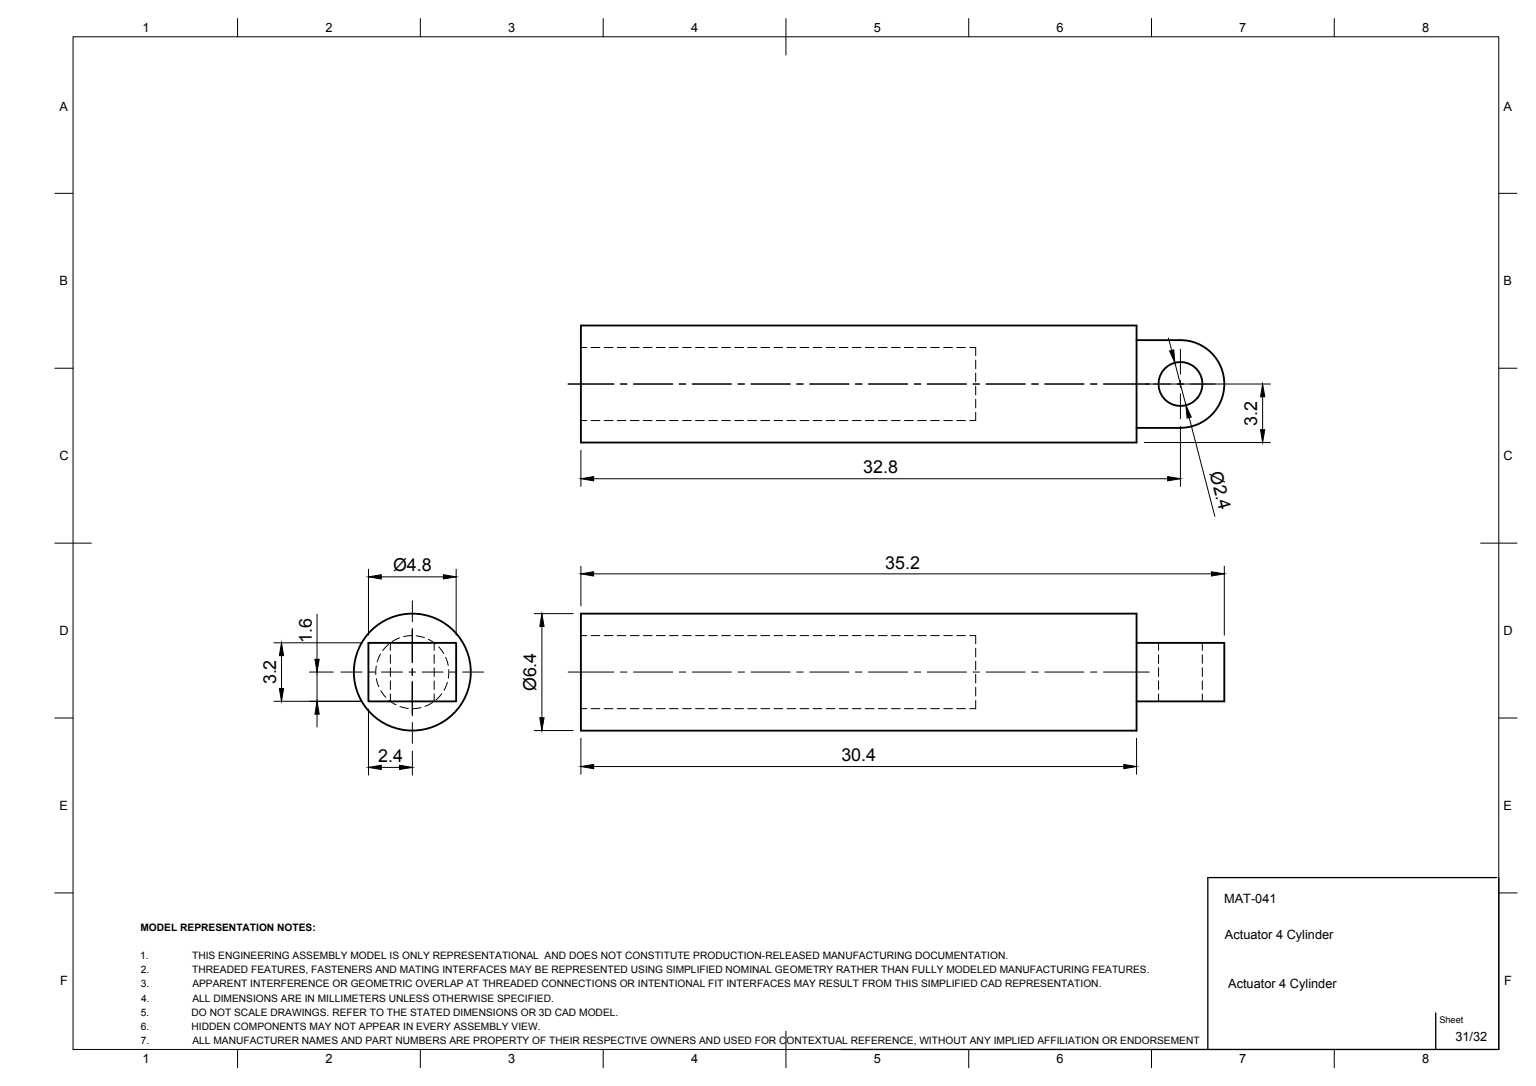
ISO-10303-21;
HEADER;
/* Generated by software containing ST-Developer
 * from STEP Tools, Inc. (www.steptools.com) 
 */

FILE_DESCRIPTION(
/* description */ ('STEP AP214'),
/* implementation_level */ '2;1');

FILE_NAME(
/* name */ 'Actuator 4 Cylinder.step',
/* time_stamp */ '2026-11-14T21:57:47-08:00',
/* author */ (''),
/* organization */ (''),
/* preprocessor_version */ 'ST-DEVELOPER v20.2',
/* originating_system */ 'Autodesk Translation Framework v15.17.0.0',
/* authorisation */ '');

FILE_SCHEMA (('AUTOMOTIVE_DESIGN { 1 0 10303 214 3 1 1 }'));
ENDSEC;

DATA;
#10=MECHANICAL_DESIGN_GEOMETRIC_PRESENTATION_REPRESENTATION('',(#264),#13199);
#228=SHAPE_REPRESENTATION_RELATIONSHIP('SRR','None',#13301,#246);
#246=ADVANCED_BREP_SHAPE_REPRESENTATION('',(#282),#13197);
#264=STYLED_ITEM('',(#13409),#282);
#282=MANIFOLD_SOLID_BREP('Body1',#6859);
#376=FACE_BOUND('',#2658,.T.);
#377=FACE_BOUND('',#2660,.T.);
#378=FACE_BOUND('',#2662,.T.);
#379=FACE_BOUND('',#2665,.T.);
#597=PLANE('',#7793);
#598=PLANE('',#7794);
#599=PLANE('',#7795);
#600=PLANE('',#7797);
#601=PLANE('',#7798);
#602=PLANE('',#7800);
#603=PLANE('',#7802);
#1103=LINE('',#13056,#1621);
#1104=LINE('',#13062,#1622);
#1105=LINE('',#13068,#1623);
#1106=LINE('',#13073,#1624);
#1107=LINE('',#13075,#1625);
#1108=LINE('',#13077,#1626);
#1109=LINE('',#13078,#1627);
#1110=LINE('',#13084,#1628);
#1111=LINE('',#13085,#1629);
#1112=LINE('',#13088,#1630);
#1113=LINE('',#13089,#1631);
#1114=LINE('',#13092,#1632);
#1115=LINE('',#13095,#1633);
#1621=VECTOR('',#9774,2.);
#1622=VECTOR('',#9781,1.2);
#1623=VECTOR('',#9788,3.2);
#1624=VECTOR('',#9793,1000.);
#1625=VECTOR('',#9794,1000.);
#1626=VECTOR('',#9795,1000.);
#1627=VECTOR('',#9796,1000.);
#1628=VECTOR('',#9803,1000.);
#1629=VECTOR('',#9804,1000.);
#1630=VECTOR('',#9807,1000.);
#1631=VECTOR('',#9808,1000.);
#1632=VECTOR('',#9811,1000.);
#1633=VECTOR('',#9816,1000.);
#1782=CYLINDRICAL_SURFACE('',#7784,2.);
#1783=CYLINDRICAL_SURFACE('',#7787,1.2);
#1784=CYLINDRICAL_SURFACE('',#7790,3.2);
#1785=CYLINDRICAL_SURFACE('',#7801,2.4);
#2171=FACE_OUTER_BOUND('',#2654,.T.);
#2172=FACE_OUTER_BOUND('',#2655,.T.);
#2173=FACE_OUTER_BOUND('',#2656,.T.);
#2174=FACE_OUTER_BOUND('',#2657,.T.);
#2175=FACE_OUTER_BOUND('',#2659,.T.);
#2176=FACE_OUTER_BOUND('',#2661,.T.);
#2177=FACE_OUTER_BOUND('',#2663,.T.);
#2178=FACE_OUTER_BOUND('',#2664,.T.);
#2179=FACE_OUTER_BOUND('',#2666,.T.);
#2180=FACE_OUTER_BOUND('',#2667,.T.);
#2181=FACE_OUTER_BOUND('',#2668,.T.);
#2654=EDGE_LOOP('',(#6364,#6365,#6366,#6367));
#2655=EDGE_LOOP('',(#6368,#6369,#6370,#6371));
#2656=EDGE_LOOP('',(#6372,#6373,#6374,#6375));
#2657=EDGE_LOOP('',(#6376));
#2658=EDGE_LOOP('',(#6377,#6378,#6379,#6380));
#2659=EDGE_LOOP('',(#6381));
#2660=EDGE_LOOP('',(#6382));
#2661=EDGE_LOOP('',(#6383,#6384,#6385,#6386));
#2662=EDGE_LOOP('',(#6387));
#2663=EDGE_LOOP('',(#6388,#6389,#6390,#6391));
#2664=EDGE_LOOP('',(#6392,#6393,#6394,#6395));
#2665=EDGE_LOOP('',(#6396));
#2666=EDGE_LOOP('',(#6397,#6398,#6399,#6400));
#2667=EDGE_LOOP('',(#6401,#6402,#6403,#6404));
#2668=EDGE_LOOP('',(#6405));
#2986=CIRCLE('',#7785,2.);
#2987=CIRCLE('',#7786,2.);
#2988=CIRCLE('',#7788,1.2);
#2989=CIRCLE('',#7789,1.2);
#2990=CIRCLE('',#7791,3.2);
#2991=CIRCLE('',#7792,3.2);
#2992=CIRCLE('',#7796,2.4);
#2993=CIRCLE('',#7799,2.4);
#3590=VERTEX_POINT('',#13053);
#3591=VERTEX_POINT('',#13055);
#3592=VERTEX_POINT('',#13059);
#3593=VERTEX_POINT('',#13061);
#3594=VERTEX_POINT('',#13065);
#3595=VERTEX_POINT('',#13067);
#3596=VERTEX_POINT('',#13071);
#3597=VERTEX_POINT('',#13072);
#3598=VERTEX_POINT('',#13074);
#3599=VERTEX_POINT('',#13076);
#3600=VERTEX_POINT('',#13081);
#3601=VERTEX_POINT('',#13082);
#3602=VERTEX_POINT('',#13087);
#3603=VERTEX_POINT('',#13091);
#4519=EDGE_CURVE('',#3590,#3590,#2986,.T.);
#4520=EDGE_CURVE('',#3590,#3591,#1103,.T.);
#4521=EDGE_CURVE('',#3591,#3591,#2987,.T.);
#4522=EDGE_CURVE('',#3592,#3592,#2988,.T.);
#4523=EDGE_CURVE('',#3592,#3593,#1104,.T.);
#4524=EDGE_CURVE('',#3593,#3593,#2989,.T.);
#4525=EDGE_CURVE('',#3594,#3594,#2990,.T.);
#4526=EDGE_CURVE('',#3594,#3595,#1105,.T.);
#4527=EDGE_CURVE('',#3595,#3595,#2991,.T.);
#4528=EDGE_CURVE('',#3596,#3597,#1106,.T.);
#4529=EDGE_CURVE('',#3598,#3596,#1107,.T.);
#4530=EDGE_CURVE('',#3599,#3598,#1108,.T.);
#4531=EDGE_CURVE('',#3597,#3599,#1109,.T.);
#4532=EDGE_CURVE('',#3600,#3601,#2992,.T.);
#4533=EDGE_CURVE('',#3601,#3596,#1110,.T.);
#4534=EDGE_CURVE('',#3600,#3597,#1111,.T.);
#4535=EDGE_CURVE('',#3602,#3599,#1112,.T.);
#4536=EDGE_CURVE('',#3602,#3600,#1113,.T.);
#4537=EDGE_CURVE('',#3603,#3598,#1114,.T.);
#4538=EDGE_CURVE('',#3603,#3602,#2993,.T.);
#4539=EDGE_CURVE('',#3601,#3603,#1115,.T.);
#6364=ORIENTED_EDGE('',*,*,#4519,.F.);
#6365=ORIENTED_EDGE('',*,*,#4520,.T.);
#6366=ORIENTED_EDGE('',*,*,#4521,.T.);
#6367=ORIENTED_EDGE('',*,*,#4520,.F.);
#6368=ORIENTED_EDGE('',*,*,#4522,.F.);
#6369=ORIENTED_EDGE('',*,*,#4523,.T.);
#6370=ORIENTED_EDGE('',*,*,#4524,.T.);
#6371=ORIENTED_EDGE('',*,*,#4523,.F.);
#6372=ORIENTED_EDGE('',*,*,#4525,.T.);
#6373=ORIENTED_EDGE('',*,*,#4526,.T.);
#6374=ORIENTED_EDGE('',*,*,#4527,.F.);
#6375=ORIENTED_EDGE('',*,*,#4526,.F.);
#6376=ORIENTED_EDGE('',*,*,#4525,.F.);
#6377=ORIENTED_EDGE('',*,*,#4528,.F.);
#6378=ORIENTED_EDGE('',*,*,#4529,.F.);
#6379=ORIENTED_EDGE('',*,*,#4530,.F.);
#6380=ORIENTED_EDGE('',*,*,#4531,.F.);
#6381=ORIENTED_EDGE('',*,*,#4527,.T.);
#6382=ORIENTED_EDGE('',*,*,#4521,.F.);
#6383=ORIENTED_EDGE('',*,*,#4532,.T.);
#6384=ORIENTED_EDGE('',*,*,#4533,.T.);
#6385=ORIENTED_EDGE('',*,*,#4528,.T.);
#6386=ORIENTED_EDGE('',*,*,#4534,.F.);
#6387=ORIENTED_EDGE('',*,*,#4522,.T.);
#6388=ORIENTED_EDGE('',*,*,#4535,.F.);
#6389=ORIENTED_EDGE('',*,*,#4536,.T.);
#6390=ORIENTED_EDGE('',*,*,#4534,.T.);
#6391=ORIENTED_EDGE('',*,*,#4531,.T.);
#6392=ORIENTED_EDGE('',*,*,#4537,.F.);
#6393=ORIENTED_EDGE('',*,*,#4538,.T.);
#6394=ORIENTED_EDGE('',*,*,#4535,.T.);
#6395=ORIENTED_EDGE('',*,*,#4530,.T.);
#6396=ORIENTED_EDGE('',*,*,#4524,.F.);
#6397=ORIENTED_EDGE('',*,*,#4533,.F.);
#6398=ORIENTED_EDGE('',*,*,#4539,.T.);
#6399=ORIENTED_EDGE('',*,*,#4537,.T.);
#6400=ORIENTED_EDGE('',*,*,#4529,.T.);
#6401=ORIENTED_EDGE('',*,*,#4536,.F.);
#6402=ORIENTED_EDGE('',*,*,#4538,.F.);
#6403=ORIENTED_EDGE('',*,*,#4539,.F.);
#6404=ORIENTED_EDGE('',*,*,#4532,.F.);
#6405=ORIENTED_EDGE('',*,*,#4519,.T.);
#6823=ADVANCED_FACE('',(#2171),#1782,.F.);
#6824=ADVANCED_FACE('',(#2172),#1783,.F.);
#6825=ADVANCED_FACE('',(#2173),#1784,.T.);
#6826=ADVANCED_FACE('',(#2174,#376),#597,.F.);
#6827=ADVANCED_FACE('',(#2175,#377),#598,.T.);
#6828=ADVANCED_FACE('',(#2176,#378),#599,.F.);
#6829=ADVANCED_FACE('',(#2177),#600,.F.);
#6830=ADVANCED_FACE('',(#2178,#379),#601,.F.);
#6831=ADVANCED_FACE('',(#2179),#602,.F.);
#6832=ADVANCED_FACE('',(#2180),#1785,.T.);
#6833=ADVANCED_FACE('',(#2181),#603,.T.);
#6859=CLOSED_SHELL('',(#6823,#6824,#6825,#6826,#6827,#6828,#6829,#6830,
#6831,#6832,#6833));
#7783=AXIS2_PLACEMENT_3D('',#13051,#9768,#9769);
#7784=AXIS2_PLACEMENT_3D('',#13052,#9770,#9771);
#7785=AXIS2_PLACEMENT_3D('',#13054,#9772,#9773);
#7786=AXIS2_PLACEMENT_3D('',#13057,#9775,#9776);
#7787=AXIS2_PLACEMENT_3D('',#13058,#9777,#9778);
#7788=AXIS2_PLACEMENT_3D('',#13060,#9779,#9780);
#7789=AXIS2_PLACEMENT_3D('',#13063,#9782,#9783);
#7790=AXIS2_PLACEMENT_3D('',#13064,#9784,#9785);
#7791=AXIS2_PLACEMENT_3D('',#13066,#9786,#9787);
#7792=AXIS2_PLACEMENT_3D('',#13069,#9789,#9790);
#7793=AXIS2_PLACEMENT_3D('',#13070,#9791,#9792);
#7794=AXIS2_PLACEMENT_3D('',#13079,#9797,#9798);
#7795=AXIS2_PLACEMENT_3D('',#13080,#9799,#9800);
#7796=AXIS2_PLACEMENT_3D('',#13083,#9801,#9802);
#7797=AXIS2_PLACEMENT_3D('',#13086,#9805,#9806);
#7798=AXIS2_PLACEMENT_3D('',#13090,#9809,#9810);
#7799=AXIS2_PLACEMENT_3D('',#13093,#9812,#9813);
#7800=AXIS2_PLACEMENT_3D('',#13094,#9814,#9815);
#7801=AXIS2_PLACEMENT_3D('',#13096,#9817,#9818);
#7802=AXIS2_PLACEMENT_3D('',#13097,#9819,#9820);
#9768=DIRECTION('axis',(0.,0.,1.));
#9769=DIRECTION('refdir',(1.,0.,0.));
#9770=DIRECTION('center_axis',(0.,0.,1.));
#9771=DIRECTION('ref_axis',(1.,0.,0.));
#9772=DIRECTION('center_axis',(0.,0.,1.));
#9773=DIRECTION('ref_axis',(1.,0.,0.));
#9774=DIRECTION('',(0.,0.,1.));
#9775=DIRECTION('center_axis',(0.,0.,1.));
#9776=DIRECTION('ref_axis',(1.,0.,0.));
#9777=DIRECTION('center_axis',(1.,-1.0842021724855E-16,0.));
#9778=DIRECTION('ref_axis',(1.0842021724855E-16,1.,0.));
#9779=DIRECTION('center_axis',(1.,-7.2280144832367E-17,0.));
#9780=DIRECTION('ref_axis',(7.2280144832367E-17,1.,0.));
#9781=DIRECTION('',(1.,-1.0842021724855E-16,0.));
#9782=DIRECTION('center_axis',(1.,-1.0842021724855E-16,0.));
#9783=DIRECTION('ref_axis',(1.0842021724855E-16,1.,0.));
#9784=DIRECTION('center_axis',(0.,0.,-1.));
#9785=DIRECTION('ref_axis',(-1.,0.,0.));
#9786=DIRECTION('center_axis',(0.,0.,1.));
#9787=DIRECTION('ref_axis',(1.,0.,0.));
#9788=DIRECTION('',(0.,0.,1.));
#9789=DIRECTION('center_axis',(0.,0.,1.));
#9790=DIRECTION('ref_axis',(1.,0.,0.));
#9791=DIRECTION('center_axis',(0.,0.,1.));
#9792=DIRECTION('ref_axis',(1.,0.,0.));
#9793=DIRECTION('',(7.2280144832367E-17,1.,0.));
#9794=DIRECTION('',(-1.,0.,0.));
#9795=DIRECTION('',(-1.44560289664734E-16,-1.,0.));
#9796=DIRECTION('',(1.,0.,0.));
#9797=DIRECTION('center_axis',(0.,0.,1.));
#9798=DIRECTION('ref_axis',(1.,0.,0.));
#9799=DIRECTION('center_axis',(1.,-7.2280144832367E-17,0.));
#9800=DIRECTION('ref_axis',(7.2280144832367E-17,1.,0.));
#9801=DIRECTION('center_axis',(-1.,7.2280144832367E-17,0.));
#9802=DIRECTION('ref_axis',(7.2280144832367E-17,1.,0.));
#9803=DIRECTION('',(0.,0.,1.));
#9804=DIRECTION('',(0.,0.,1.));
#9805=DIRECTION('center_axis',(0.,-1.,0.));
#9806=DIRECTION('ref_axis',(0.,0.,-1.));
#9807=DIRECTION('',(0.,0.,1.));
#9808=DIRECTION('',(-1.,0.,0.));
#9809=DIRECTION('center_axis',(-1.,1.44560289664734E-16,0.));
#9810=DIRECTION('ref_axis',(-1.44560289664734E-16,-1.,0.));
#9811=DIRECTION('',(0.,0.,1.));
#9812=DIRECTION('center_axis',(1.,-1.44560289664734E-16,0.));
#9813=DIRECTION('ref_axis',(-1.44560289664734E-16,-1.,0.));
#9814=DIRECTION('center_axis',(0.,1.,0.));
#9815=DIRECTION('ref_axis',(0.,0.,1.));
#9816=DIRECTION('',(1.,0.,0.));
#9817=DIRECTION('center_axis',(-1.,0.,0.));
#9818=DIRECTION('ref_axis',(0.,1.22464679914735E-16,-1.));
#9819=DIRECTION('center_axis',(0.,0.,1.));
#9820=DIRECTION('ref_axis',(1.,0.,0.));
#13051=CARTESIAN_POINT('',(0.,0.,0.));
#13052=CARTESIAN_POINT('Origin',(3.77881193895716E-17,0.,11.9128278522764));
#13053=CARTESIAN_POINT('',(-2.,-2.44929359829471E-16,11.9128278522764));
#13054=CARTESIAN_POINT('Origin',(3.77881193895716E-17,0.,11.9128278522764));
#13055=CARTESIAN_POINT('',(-2.,-2.44929359829471E-16,33.5128278522764));
#13056=CARTESIAN_POINT('',(-2.,-2.44929359829471E-16,11.9128278522764));
#13057=CARTESIAN_POINT('Origin',(3.77881193895716E-17,0.,33.5128278522764));
#13058=CARTESIAN_POINT('Origin',(-3.2,4.19224840027728E-16,0.712827852276406));
#13059=CARTESIAN_POINT('',(-1.6,-1.2,0.712827852276406));
#13060=CARTESIAN_POINT('Origin',(-1.6,2.45752492430048E-16,0.712827852276406));
#13061=CARTESIAN_POINT('',(1.6,-1.2,0.712827852276406));
#13062=CARTESIAN_POINT('',(-3.2,-1.2,0.712827852276406));
#13063=CARTESIAN_POINT('Origin',(1.6,-1.01192202765314E-16,0.712827852276406));
#13064=CARTESIAN_POINT('Origin',(3.77881193895716E-17,0.,33.5128278522764));
#13065=CARTESIAN_POINT('',(3.2,-3.91886975727153E-16,3.11282785227641));
#13066=CARTESIAN_POINT('Origin',(3.77881193895716E-17,0.,3.11282785227641));
#13067=CARTESIAN_POINT('',(3.2,-3.91886975727153E-16,33.5128278522764));
#13068=CARTESIAN_POINT('',(3.2,-3.91886975727153E-16,33.5128278522764));
#13069=CARTESIAN_POINT('Origin',(3.77881193895716E-17,0.,33.5128278522764));
#13070=CARTESIAN_POINT('Origin',(3.77881193895716E-17,0.,3.11282785227641));
#13071=CARTESIAN_POINT('',(-1.6,-2.4,3.11282785227641));
#13072=CARTESIAN_POINT('',(-1.6,2.4,3.11282785227641));
#13073=CARTESIAN_POINT('',(-1.6,2.4,3.11282785227641));
#13074=CARTESIAN_POINT('',(1.6,-2.4,3.11282785227641));
#13075=CARTESIAN_POINT('',(1.6,-2.4,3.11282785227641));
#13076=CARTESIAN_POINT('',(1.6,2.4,3.11282785227641));
#13077=CARTESIAN_POINT('',(1.6,2.4,3.11282785227641));
#13078=CARTESIAN_POINT('',(1.6,2.4,3.11282785227641));
#13079=CARTESIAN_POINT('Origin',(3.77881193895716E-17,0.,33.5128278522764));
#13080=CARTESIAN_POINT('Origin',(-1.6,2.4,-1.68717214772359));
#13081=CARTESIAN_POINT('',(-1.6,2.4,0.712827852276406));
#13082=CARTESIAN_POINT('',(-1.6,-2.4,0.712827852276406));
#13083=CARTESIAN_POINT('Origin',(-1.6,0.,0.712827852276406));
#13084=CARTESIAN_POINT('',(-1.6,-2.4,-1.68717214772359));
#13085=CARTESIAN_POINT('',(-1.6,2.4,-1.68717214772359));
#13086=CARTESIAN_POINT('Origin',(1.6,2.4,-1.68717214772359));
#13087=CARTESIAN_POINT('',(1.6,2.4,0.712827852276406));
#13088=CARTESIAN_POINT('',(1.6,2.4,-1.68717214772359));
#13089=CARTESIAN_POINT('',(-1.6,2.4,0.712827852276406));
#13090=CARTESIAN_POINT('Origin',(1.6,2.4,-1.68717214772359));
#13091=CARTESIAN_POINT('',(1.6,-2.4,0.712827852276406));
#13092=CARTESIAN_POINT('',(1.6,-2.4,-1.68717214772359));
#13093=CARTESIAN_POINT('Origin',(1.6,0.,0.712827852276406));
#13094=CARTESIAN_POINT('Origin',(1.6,-2.4,-1.68717214772359));
#13095=CARTESIAN_POINT('',(1.6,-2.4,0.712827852276406));
#13096=CARTESIAN_POINT('Origin',(3.77881193895716E-17,0.,0.712827852276406));
#13097=CARTESIAN_POINT('Origin',(3.77881193895716E-17,0.,11.9128278522764));
#13171=UNCERTAINTY_MEASURE_WITH_UNIT(LENGTH_MEASURE(0.01),#13200,
'DISTANCE_ACCURACY_VALUE',
'Maximum model space distance between geometric entities at asserted c
onnectivities');
#13173=UNCERTAINTY_MEASURE_WITH_UNIT(LENGTH_MEASURE(0.01),#13200,
'DISTANCE_ACCURACY_VALUE',
'Maximum model space distance between geometric entities at asserted c
onnectivities');
#13197=(
GEOMETRIC_REPRESENTATION_CONTEXT(3)
GLOBAL_UNCERTAINTY_ASSIGNED_CONTEXT((#13171))
GLOBAL_UNIT_ASSIGNED_CONTEXT((#13200,#13202,#13203))
REPRESENTATION_CONTEXT('','3D')
);
#13199=(
GEOMETRIC_REPRESENTATION_CONTEXT(3)
GLOBAL_UNCERTAINTY_ASSIGNED_CONTEXT((#13173))
GLOBAL_UNIT_ASSIGNED_CONTEXT((#13200,#13202,#13203))
REPRESENTATION_CONTEXT('','3D')
);
#13200=(
LENGTH_UNIT()
NAMED_UNIT(*)
SI_UNIT(.MILLI.,.METRE.)
);
#13202=(
NAMED_UNIT(*)
PLANE_ANGLE_UNIT()
SI_UNIT($,.RADIAN.)
);
#13203=(
NAMED_UNIT(*)
SI_UNIT($,.STERADIAN.)
SOLID_ANGLE_UNIT()
);
#13227=SHAPE_DEFINITION_REPRESENTATION(#13266,#13301);
#13266=PRODUCT_DEFINITION_SHAPE('',$,#13327);
#13301=SHAPE_REPRESENTATION('',(#7783),#13197);
#13303=PRODUCT_DEFINITION_CONTEXT('part definition',#13380,'design');
#13327=PRODUCT_DEFINITION('Actuator 4 Cylinder','Actuator 4 Cylinder',#13352,
#13303);
#13352=PRODUCT_DEFINITION_FORMATION('',$,#13405);
#13380=APPLICATION_CONTEXT(
'Core Data for Automotive Mechanical Design Process');
#13381=PRODUCT_CONTEXT('part definition',#13380,'mechanical');
#13405=PRODUCT('Actuator 4 Cylinder','Actuator 4 Cylinder',$,(#13381));
#13409=PRESENTATION_STYLE_ASSIGNMENT((#13414));
#13414=SURFACE_STYLE_USAGE(.BOTH.,#13419);
#13419=SURFACE_SIDE_STYLE('',(#13424));
#13424=SURFACE_STYLE_FILL_AREA(#13429);
#13429=FILL_AREA_STYLE('Opaque(61,176,222)',(#13434));
#13434=FILL_AREA_STYLE_COLOUR('Opaque(61,176,222)',#13439);
#13439=COLOUR_RGB('Opaque(61,176,222)',0.23921568627451,0.690196078431373,
0.870588235294118);
ENDSEC;
END-ISO-10303-21;
